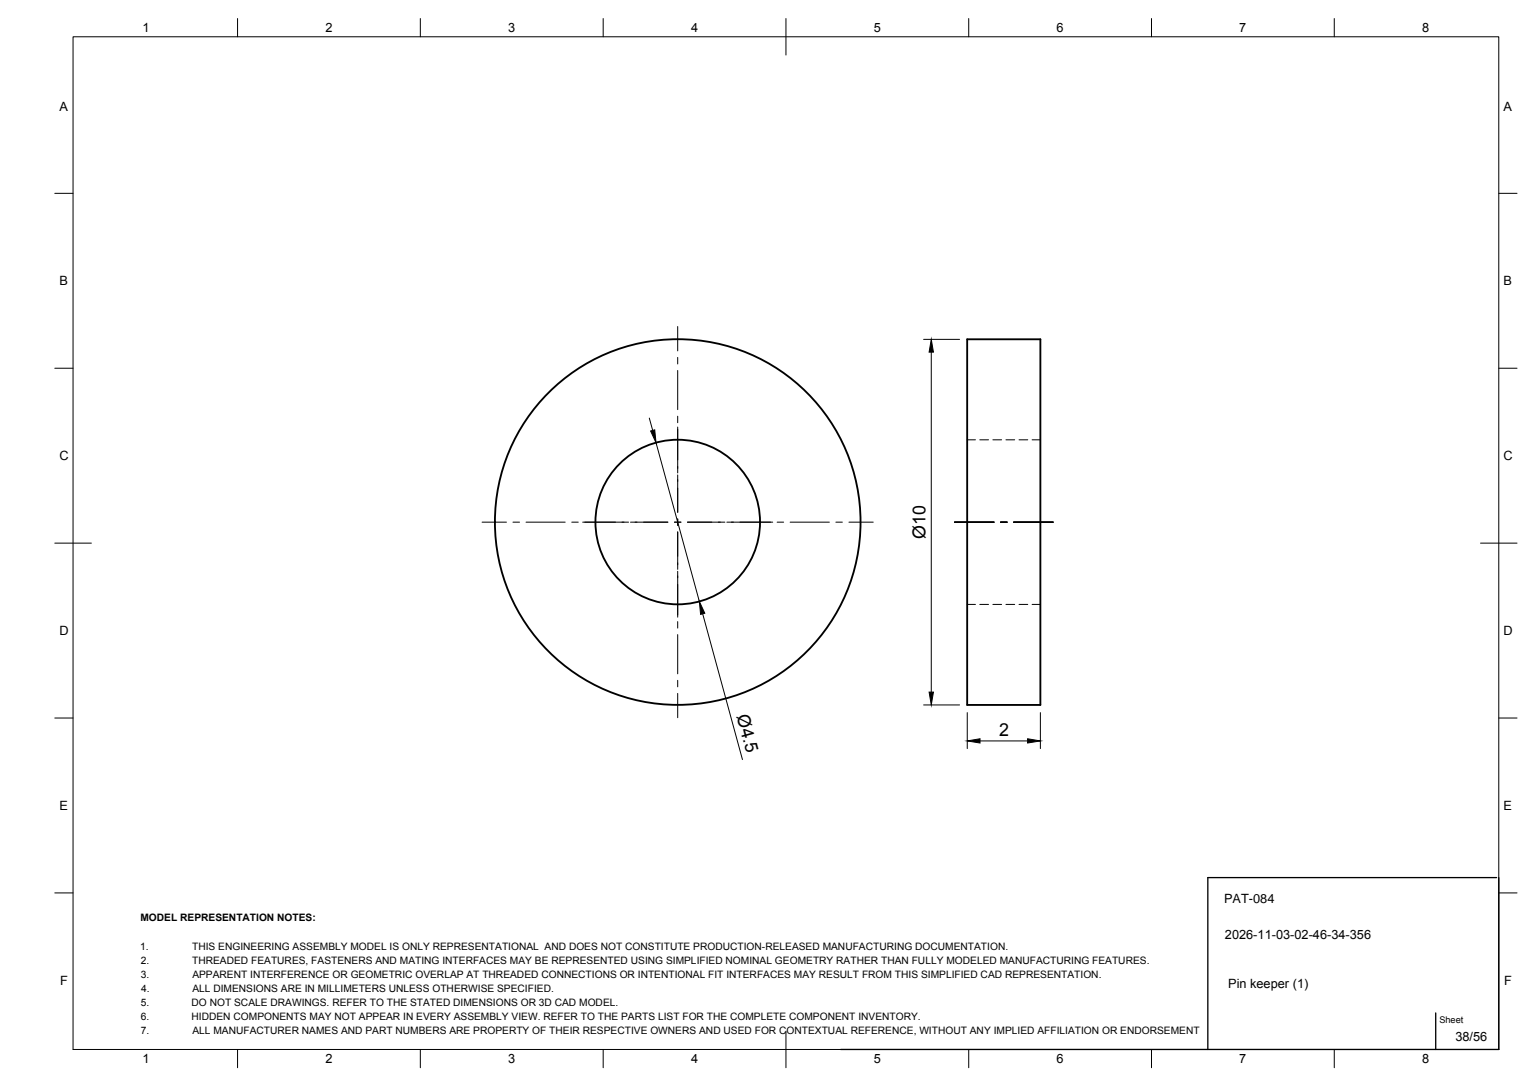
ISO-10303-21;
HEADER;
/* Generated by software containing ST-Developer
 * from STEP Tools, Inc. (www.steptools.com) 
 */

FILE_DESCRIPTION(
/* description */ ('Quick-return (Whitworth) mechanism'),
/* implementation_level */ '2;1');

FILE_NAME(
/* name */ 'Pin keeper (1).step',
/* time_stamp */ '2026-10-28T03:25:57-07:00',
/* author */ (''),
/* organization */ (''),
/* preprocessor_version */ 'ST-DEVELOPER v20.2',
/* originating_system */ 'Autodesk Translation Framework v15.17.0.0',
/* authorisation */ '');

FILE_SCHEMA (('AUTOMOTIVE_DESIGN { 1 0 10303 214 3 1 1 }'));
ENDSEC;

DATA;
#10=MECHANICAL_DESIGN_GEOMETRIC_PRESENTATION_REPRESENTATION('',(#526),#14878);
#430=SHAPE_REPRESENTATION_RELATIONSHIP('SRR','None',#15101,#474);
#474=ADVANCED_BREP_SHAPE_REPRESENTATION('',(#577),#14858);
#526=STYLED_ITEM('',(#15406),#577);
#577=MANIFOLD_SOLID_BREP('Body1',#7881);
#744=FACE_BOUND('',#1983,.T.);
#745=FACE_BOUND('',#1985,.T.);
#937=PLANE('',#9073);
#938=PLANE('',#9074);
#1361=FACE_OUTER_BOUND('',#1980,.T.);
#1362=FACE_OUTER_BOUND('',#1981,.T.);
#1363=FACE_OUTER_BOUND('',#1982,.T.);
#1364=FACE_OUTER_BOUND('',#1984,.T.);
#1980=EDGE_LOOP('',(#6540,#6541,#6542,#6543));
#1981=EDGE_LOOP('',(#6544,#6545,#6546,#6547));
#1982=EDGE_LOOP('',(#6548));
#1983=EDGE_LOOP('',(#6549));
#1984=EDGE_LOOP('',(#6550));
#1985=EDGE_LOOP('',(#6551));
#2443=LINE('',#13974,#2966);
#2444=LINE('',#13980,#2967);
#2966=VECTOR('',#11040,0.225);
#2967=VECTOR('',#11047,0.5);
#3546=CIRCLE('',#9068,0.225);
#3547=CIRCLE('',#9069,0.225);
#3548=CIRCLE('',#9071,0.5);
#3549=CIRCLE('',#9072,0.5);
#4067=VERTEX_POINT('',#13971);
#4068=VERTEX_POINT('',#13973);
#4069=VERTEX_POINT('',#13977);
#4070=VERTEX_POINT('',#13979);
#4927=EDGE_CURVE('',#4067,#4067,#3546,.T.);
#4928=EDGE_CURVE('',#4067,#4068,#2443,.T.);
#4929=EDGE_CURVE('',#4068,#4068,#3547,.T.);
#4930=EDGE_CURVE('',#4069,#4069,#3548,.T.);
#4931=EDGE_CURVE('',#4069,#4070,#2444,.T.);
#4932=EDGE_CURVE('',#4070,#4070,#3549,.T.);
#6540=ORIENTED_EDGE('',*,*,#4927,.F.);
#6541=ORIENTED_EDGE('',*,*,#4928,.T.);
#6542=ORIENTED_EDGE('',*,*,#4929,.T.);
#6543=ORIENTED_EDGE('',*,*,#4928,.F.);
#6544=ORIENTED_EDGE('',*,*,#4930,.F.);
#6545=ORIENTED_EDGE('',*,*,#4931,.T.);
#6546=ORIENTED_EDGE('',*,*,#4932,.T.);
#6547=ORIENTED_EDGE('',*,*,#4931,.F.);
#6548=ORIENTED_EDGE('',*,*,#4930,.T.);
#6549=ORIENTED_EDGE('',*,*,#4927,.T.);
#6550=ORIENTED_EDGE('',*,*,#4932,.F.);
#6551=ORIENTED_EDGE('',*,*,#4929,.F.);
#7343=CYLINDRICAL_SURFACE('',#9067,0.225);
#7344=CYLINDRICAL_SURFACE('',#9070,0.5);
#7692=ADVANCED_FACE('',(#1361),#7343,.F.);
#7693=ADVANCED_FACE('',(#1362),#7344,.T.);
#7694=ADVANCED_FACE('',(#1363,#744),#937,.T.);
#7695=ADVANCED_FACE('',(#1364,#745),#938,.F.);
#7881=CLOSED_SHELL('',(#7692,#7693,#7694,#7695));
#9066=AXIS2_PLACEMENT_3D('',#13969,#11034,#11035);
#9067=AXIS2_PLACEMENT_3D('',#13970,#11036,#11037);
#9068=AXIS2_PLACEMENT_3D('',#13972,#11038,#11039);
#9069=AXIS2_PLACEMENT_3D('',#13975,#11041,#11042);
#9070=AXIS2_PLACEMENT_3D('',#13976,#11043,#11044);
#9071=AXIS2_PLACEMENT_3D('',#13978,#11045,#11046);
#9072=AXIS2_PLACEMENT_3D('',#13981,#11048,#11049);
#9073=AXIS2_PLACEMENT_3D('',#13982,#11050,#11051);
#9074=AXIS2_PLACEMENT_3D('',#13983,#11052,#11053);
#11034=DIRECTION('axis',(0.,0.,1.));
#11035=DIRECTION('refdir',(1.,0.,0.));
#11036=DIRECTION('center_axis',(0.,0.,1.));
#11037=DIRECTION('ref_axis',(1.,0.,0.));
#11038=DIRECTION('center_axis',(0.,0.,-1.));
#11039=DIRECTION('ref_axis',(1.,0.,0.));
#11040=DIRECTION('',(0.,0.,-1.));
#11041=DIRECTION('center_axis',(0.,0.,-1.));
#11042=DIRECTION('ref_axis',(1.,0.,0.));
#11043=DIRECTION('center_axis',(0.,0.,1.));
#11044=DIRECTION('ref_axis',(1.,0.,0.));
#11045=DIRECTION('center_axis',(0.,0.,1.));
#11046=DIRECTION('ref_axis',(1.,0.,0.));
#11047=DIRECTION('',(0.,0.,-1.));
#11048=DIRECTION('center_axis',(0.,0.,1.));
#11049=DIRECTION('ref_axis',(1.,0.,0.));
#11050=DIRECTION('center_axis',(0.,0.,1.));
#11051=DIRECTION('ref_axis',(1.,0.,0.));
#11052=DIRECTION('center_axis',(0.,0.,1.));
#11053=DIRECTION('ref_axis',(1.,0.,0.));
#13969=CARTESIAN_POINT('',(0.,0.,0.));
#13970=CARTESIAN_POINT('Origin',(0.,12.,9.8));
#13971=CARTESIAN_POINT('',(-0.225,12.,10.));
#13972=CARTESIAN_POINT('Origin',(0.,12.,10.));
#13973=CARTESIAN_POINT('',(-0.225,12.,9.8));
#13974=CARTESIAN_POINT('',(-0.225,12.,9.8));
#13975=CARTESIAN_POINT('Origin',(0.,12.,9.8));
#13976=CARTESIAN_POINT('Origin',(0.,12.,9.8));
#13977=CARTESIAN_POINT('',(-0.5,12.,10.));
#13978=CARTESIAN_POINT('Origin',(0.,12.,10.));
#13979=CARTESIAN_POINT('',(-0.5,12.,9.8));
#13980=CARTESIAN_POINT('',(-0.5,12.,9.8));
#13981=CARTESIAN_POINT('Origin',(0.,12.,9.8));
#13982=CARTESIAN_POINT('Origin',(0.,12.,10.));
#13983=CARTESIAN_POINT('Origin',(0.,12.,9.8));
#14804=UNCERTAINTY_MEASURE_WITH_UNIT(LENGTH_MEASURE(0.001),#14879,
'DISTANCE_ACCURACY_VALUE',
'Maximum model space distance between geometric entities at asserted c
onnectivities');
#14824=UNCERTAINTY_MEASURE_WITH_UNIT(LENGTH_MEASURE(0.001),#14879,
'DISTANCE_ACCURACY_VALUE',
'Maximum model space distance between geometric entities at asserted c
onnectivities');
#14858=(
GEOMETRIC_REPRESENTATION_CONTEXT(3)
GLOBAL_UNCERTAINTY_ASSIGNED_CONTEXT((#14804))
GLOBAL_UNIT_ASSIGNED_CONTEXT((#14879,#14881,#14882))
REPRESENTATION_CONTEXT('','3D')
);
#14878=(
GEOMETRIC_REPRESENTATION_CONTEXT(3)
GLOBAL_UNCERTAINTY_ASSIGNED_CONTEXT((#14824))
GLOBAL_UNIT_ASSIGNED_CONTEXT((#14879,#14881,#14882))
REPRESENTATION_CONTEXT('','3D')
);
#14879=(
LENGTH_UNIT()
NAMED_UNIT(*)
SI_UNIT(.CENTI.,.METRE.)
);
#14881=(
NAMED_UNIT(*)
PLANE_ANGLE_UNIT()
SI_UNIT($,.RADIAN.)
);
#14882=(
NAMED_UNIT(*)
SI_UNIT($,.STERADIAN.)
SOLID_ANGLE_UNIT()
);
#14916=SHAPE_DEFINITION_REPRESENTATION(#14974,#15101);
#14974=PRODUCT_DEFINITION_SHAPE('',$,#15155);
#15101=SHAPE_REPRESENTATION('',(#9066),#14858);
#15121=PRODUCT_DEFINITION_CONTEXT('part definition',#15282,'design');
#15155=PRODUCT_DEFINITION('Pin keeper (1)','Pin keeper (1)',#15208,#15121);
#15208=PRODUCT_DEFINITION_FORMATION('',$,#15317);
#15282=APPLICATION_CONTEXT(
'Core Data for Automotive Mechanical Design Process');
#15283=PRODUCT_CONTEXT('part definition',#15282,'mechanical');
#15317=PRODUCT('Pin keeper (1)','Pin keeper (1)','Pin keeper (1)',(#15283));
#15400=COLOUR_RGB('Grey',0.48,0.52,0.57);
#15401=FILL_AREA_STYLE_COLOUR('',#15400);
#15402=FILL_AREA_STYLE('',(#15401));
#15403=SURFACE_STYLE_FILL_AREA(#15402);
#15404=SURFACE_SIDE_STYLE('',(#15403));
#15405=SURFACE_STYLE_USAGE(.BOTH.,#15404);
#15406=PRESENTATION_STYLE_ASSIGNMENT((#15405));
ENDSEC;
END-ISO-10303-21;
